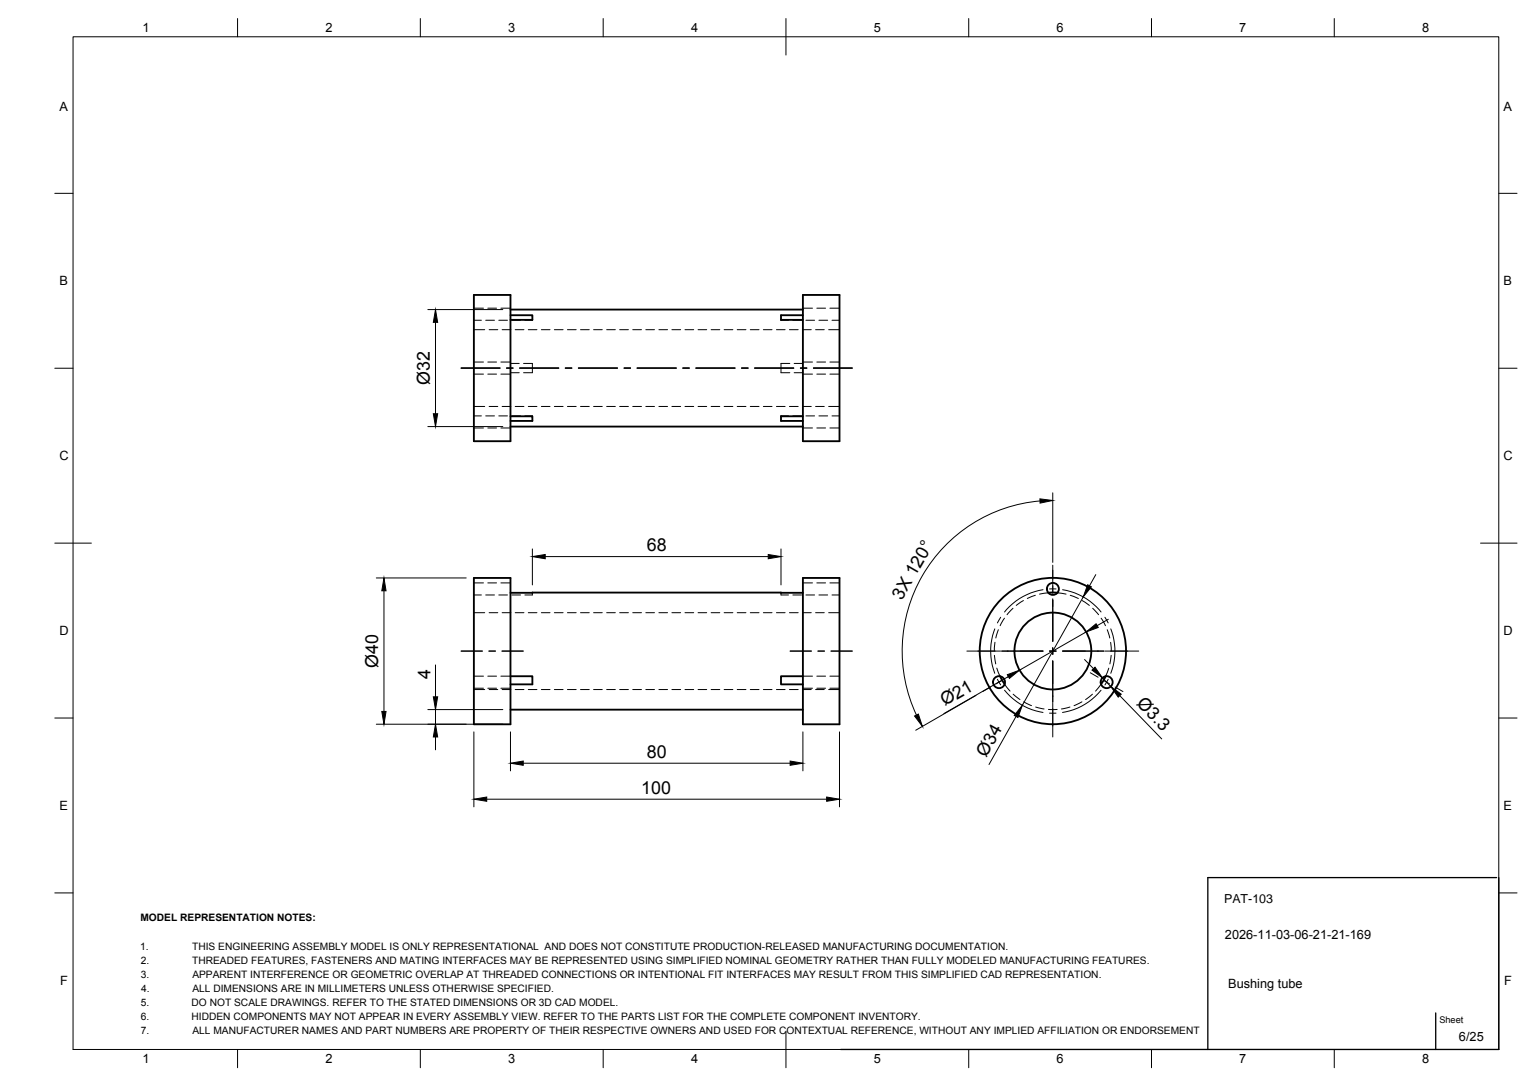
ISO-10303-21;
HEADER;
/* Generated by software containing ST-Developer
 * from STEP Tools, Inc. (www.steptools.com) 
 */

FILE_DESCRIPTION(
/* description */ ('Telescoping shaft support with lock collar'),
/* implementation_level */ '2;1');

FILE_NAME(
/* name */ 'Bushing tube.step',
/* time_stamp */ '2026-10-27T10:48:51-07:00',
/* author */ (''),
/* organization */ (''),
/* preprocessor_version */ 'ST-DEVELOPER v20.2',
/* originating_system */ 'Autodesk Translation Framework v15.17.0.0',
/* authorisation */ '');

FILE_SCHEMA (('AUTOMOTIVE_DESIGN { 1 0 10303 214 3 1 1 }'));
ENDSEC;

DATA;
#10=MECHANICAL_DESIGN_GEOMETRIC_PRESENTATION_REPRESENTATION('',(#242),#7349);
#202=SHAPE_REPRESENTATION_RELATIONSHIP('SRR','None',#7444,#222);
#222=ADVANCED_BREP_SHAPE_REPRESENTATION('',(#262),#7328);
#242=STYLED_ITEM('',(#7641),#262);
#262=MANIFOLD_SOLID_BREP('Body1',#3965);
#287=FACE_BOUND('',#746,.T.);
#288=FACE_BOUND('',#756,.T.);
#289=FACE_BOUND('',#760,.T.);
#290=FACE_BOUND('',#761,.T.);
#291=FACE_BOUND('',#762,.T.);
#292=FACE_BOUND('',#763,.T.);
#293=FACE_BOUND('',#765,.T.);
#294=FACE_BOUND('',#766,.T.);
#295=FACE_BOUND('',#767,.T.);
#296=FACE_BOUND('',#768,.T.);
#365=PLANE('',#4234);
#366=PLANE('',#4242);
#367=PLANE('',#4249);
#368=PLANE('',#4251);
#369=PLANE('',#4256);
#370=PLANE('',#4264);
#371=PLANE('',#4271);
#372=PLANE('',#4284);
#373=PLANE('',#4291);
#374=PLANE('',#4292);
#505=FACE_OUTER_BOUND('',#739,.T.);
#506=FACE_OUTER_BOUND('',#740,.T.);
#507=FACE_OUTER_BOUND('',#741,.T.);
#508=FACE_OUTER_BOUND('',#742,.T.);
#509=FACE_OUTER_BOUND('',#743,.T.);
#510=FACE_OUTER_BOUND('',#744,.T.);
#511=FACE_OUTER_BOUND('',#745,.T.);
#512=FACE_OUTER_BOUND('',#747,.T.);
#513=FACE_OUTER_BOUND('',#748,.T.);
#514=FACE_OUTER_BOUND('',#749,.T.);
#515=FACE_OUTER_BOUND('',#750,.T.);
#516=FACE_OUTER_BOUND('',#751,.T.);
#517=FACE_OUTER_BOUND('',#752,.T.);
#518=FACE_OUTER_BOUND('',#753,.T.);
#519=FACE_OUTER_BOUND('',#754,.T.);
#520=FACE_OUTER_BOUND('',#755,.T.);
#521=FACE_OUTER_BOUND('',#757,.T.);
#522=FACE_OUTER_BOUND('',#758,.T.);
#523=FACE_OUTER_BOUND('',#759,.T.);
#524=FACE_OUTER_BOUND('',#764,.T.);
#739=EDGE_LOOP('',(#2690,#2691,#2692,#2693,#2694,#2695,#2696,#2697));
#740=EDGE_LOOP('',(#2698,#2699,#2700));
#741=EDGE_LOOP('',(#2701,#2702,#2703,#2704,#2705,#2706,#2707,#2708));
#742=EDGE_LOOP('',(#2709,#2710));
#743=EDGE_LOOP('',(#2711,#2712,#2713,#2714,#2715,#2716,#2717,#2718));
#744=EDGE_LOOP('',(#2719,#2720));
#745=EDGE_LOOP('',(#2721));
#746=EDGE_LOOP('',(#2722,#2723,#2724,#2725,#2726,#2727,#2728,#2729,#2730));
#747=EDGE_LOOP('',(#2731,#2732,#2733));
#748=EDGE_LOOP('',(#2734,#2735,#2736,#2737,#2738,#2739,#2740,#2741));
#749=EDGE_LOOP('',(#2742,#2743));
#750=EDGE_LOOP('',(#2744,#2745,#2746,#2747,#2748,#2749,#2750,#2751));
#751=EDGE_LOOP('',(#2752,#2753));
#752=EDGE_LOOP('',(#2754,#2755,#2756,#2757,#2758,#2759,#2760,#2761));
#753=EDGE_LOOP('',(#2762,#2763,#2764,#2765,#2766,#2767,#2768,#2769,#2770,
#2771,#2772,#2773,#2774,#2775,#2776,#2777,#2778,#2779,#2780,#2781,#2782,
#2783,#2784,#2785,#2786,#2787,#2788,#2789));
#754=EDGE_LOOP('',(#2790,#2791,#2792,#2793));
#755=EDGE_LOOP('',(#2794));
#756=EDGE_LOOP('',(#2795,#2796,#2797,#2798,#2799,#2800,#2801,#2802,#2803));
#757=EDGE_LOOP('',(#2804,#2805,#2806,#2807));
#758=EDGE_LOOP('',(#2808,#2809,#2810,#2811));
#759=EDGE_LOOP('',(#2812));
#760=EDGE_LOOP('',(#2813));
#761=EDGE_LOOP('',(#2814));
#762=EDGE_LOOP('',(#2815));
#763=EDGE_LOOP('',(#2816));
#764=EDGE_LOOP('',(#2817));
#765=EDGE_LOOP('',(#2818));
#766=EDGE_LOOP('',(#2819));
#767=EDGE_LOOP('',(#2820));
#768=EDGE_LOOP('',(#2821));
#1043=LINE('',#6044,#1323);
#1044=LINE('',#6048,#1324);
#1045=LINE('',#6052,#1325);
#1046=LINE('',#6062,#1326);
#1047=LINE('',#6066,#1327);
#1048=LINE('',#6070,#1328);
#1049=LINE('',#6078,#1329);
#1050=LINE('',#6082,#1330);
#1051=LINE('',#6086,#1331);
#1052=LINE('',#6108,#1332);
#1053=LINE('',#6111,#1333);
#1054=LINE('',#6113,#1334);
#1055=LINE('',#6124,#1335);
#1056=LINE('',#6127,#1336);
#1057=LINE('',#6129,#1337);
#1058=LINE('',#6140,#1338);
#1059=LINE('',#6143,#1339);
#1060=LINE('',#6145,#1340);
#1061=LINE('',#6148,#1341);
#1062=LINE('',#6155,#1342);
#1063=LINE('',#6161,#1343);
#1064=LINE('',#6167,#1344);
#1323=VECTOR('',#4769,1.);
#1324=VECTOR('',#4772,1.);
#1325=VECTOR('',#4775,0.165);
#1326=VECTOR('',#4788,1.);
#1327=VECTOR('',#4791,1.);
#1328=VECTOR('',#4794,0.165);
#1329=VECTOR('',#4805,1.);
#1330=VECTOR('',#4808,1.);
#1331=VECTOR('',#4811,0.165);
#1332=VECTOR('',#4842,0.165);
#1333=VECTOR('',#4845,1.);
#1334=VECTOR('',#4846,1.);
#1335=VECTOR('',#4859,0.165);
#1336=VECTOR('',#4862,1.);
#1337=VECTOR('',#4863,1.);
#1338=VECTOR('',#4876,0.165);
#1339=VECTOR('',#4879,1.);
#1340=VECTOR('',#4880,1.);
#1341=VECTOR('',#4885,1.6);
#1342=VECTOR('',#4896,2.);
#1343=VECTOR('',#4903,2.);
#1344=VECTOR('',#4910,1.05);
#1595=CIRCLE('',#4230,0.165);
#1596=CIRCLE('',#4231,0.165);
#1597=CIRCLE('',#4232,0.165);
#1598=CIRCLE('',#4233,0.165);
#1599=CIRCLE('',#4235,1.6);
#1600=CIRCLE('',#4236,1.6);
#1601=CIRCLE('',#4238,0.165);
#1602=CIRCLE('',#4239,0.165);
#1603=CIRCLE('',#4240,0.165);
#1604=CIRCLE('',#4241,0.165);
#1605=CIRCLE('',#4243,1.6);
#1606=CIRCLE('',#4245,0.165);
#1607=CIRCLE('',#4246,0.165);
#1608=CIRCLE('',#4247,0.165);
#1609=CIRCLE('',#4248,0.165);
#1610=CIRCLE('',#4250,1.6);
#1611=CIRCLE('',#4252,2.);
#1612=CIRCLE('',#4253,1.6);
#1613=CIRCLE('',#4254,1.6);
#1614=CIRCLE('',#4255,1.6);
#1615=CIRCLE('',#4257,1.6);
#1616=CIRCLE('',#4258,0.165);
#1617=CIRCLE('',#4259,1.6);
#1618=CIRCLE('',#4261,0.165);
#1619=CIRCLE('',#4262,0.165);
#1620=CIRCLE('',#4263,0.165);
#1621=CIRCLE('',#4265,1.6);
#1622=CIRCLE('',#4266,0.165);
#1623=CIRCLE('',#4268,0.165);
#1624=CIRCLE('',#4269,0.165);
#1625=CIRCLE('',#4270,0.165);
#1626=CIRCLE('',#4272,1.6);
#1627=CIRCLE('',#4273,0.165);
#1628=CIRCLE('',#4275,0.165);
#1629=CIRCLE('',#4276,0.165);
#1630=CIRCLE('',#4277,0.165);
#1631=CIRCLE('',#4279,1.6);
#1632=CIRCLE('',#4280,1.6);
#1633=CIRCLE('',#4281,1.6);
#1634=CIRCLE('',#4283,2.);
#1635=CIRCLE('',#4285,2.);
#1636=CIRCLE('',#4287,2.);
#1637=CIRCLE('',#4289,1.05);
#1638=CIRCLE('',#4290,1.05);
#1814=VERTEX_POINT('',#6042);
#1815=VERTEX_POINT('',#6043);
#1816=VERTEX_POINT('',#6045);
#1817=VERTEX_POINT('',#6047);
#1818=VERTEX_POINT('',#6049);
#1819=VERTEX_POINT('',#6051);
#1820=VERTEX_POINT('',#6056);
#1821=VERTEX_POINT('',#6060);
#1822=VERTEX_POINT('',#6061);
#1823=VERTEX_POINT('',#6063);
#1824=VERTEX_POINT('',#6065);
#1825=VERTEX_POINT('',#6067);
#1826=VERTEX_POINT('',#6069);
#1827=VERTEX_POINT('',#6076);
#1828=VERTEX_POINT('',#6077);
#1829=VERTEX_POINT('',#6079);
#1830=VERTEX_POINT('',#6081);
#1831=VERTEX_POINT('',#6083);
#1832=VERTEX_POINT('',#6085);
#1833=VERTEX_POINT('',#6092);
#1834=VERTEX_POINT('',#6098);
#1835=VERTEX_POINT('',#6099);
#1836=VERTEX_POINT('',#6101);
#1837=VERTEX_POINT('',#6105);
#1838=VERTEX_POINT('',#6107);
#1839=VERTEX_POINT('',#6109);
#1840=VERTEX_POINT('',#6112);
#1841=VERTEX_POINT('',#6116);
#1842=VERTEX_POINT('',#6117);
#1843=VERTEX_POINT('',#6121);
#1844=VERTEX_POINT('',#6123);
#1845=VERTEX_POINT('',#6125);
#1846=VERTEX_POINT('',#6128);
#1847=VERTEX_POINT('',#6132);
#1848=VERTEX_POINT('',#6133);
#1849=VERTEX_POINT('',#6137);
#1850=VERTEX_POINT('',#6139);
#1851=VERTEX_POINT('',#6141);
#1852=VERTEX_POINT('',#6144);
#1853=VERTEX_POINT('',#6153);
#1854=VERTEX_POINT('',#6157);
#1855=VERTEX_POINT('',#6160);
#1856=VERTEX_POINT('',#6164);
#1857=VERTEX_POINT('',#6166);
#2157=EDGE_CURVE('',#1814,#1815,#1043,.T.);
#2158=EDGE_CURVE('',#1816,#1814,#1595,.T.);
#2159=EDGE_CURVE('',#1817,#1816,#1044,.T.);
#2160=EDGE_CURVE('',#1818,#1817,#1596,.T.);
#2161=EDGE_CURVE('',#1818,#1819,#1045,.T.);
#2162=EDGE_CURVE('',#1819,#1819,#1597,.T.);
#2163=EDGE_CURVE('',#1815,#1818,#1598,.T.);
#2164=EDGE_CURVE('',#1816,#1820,#1599,.T.);
#2165=EDGE_CURVE('',#1820,#1814,#1600,.T.);
#2166=EDGE_CURVE('',#1821,#1822,#1046,.T.);
#2167=EDGE_CURVE('',#1823,#1821,#1601,.T.);
#2168=EDGE_CURVE('',#1824,#1823,#1047,.T.);
#2169=EDGE_CURVE('',#1825,#1824,#1602,.T.);
#2170=EDGE_CURVE('',#1825,#1826,#1048,.T.);
#2171=EDGE_CURVE('',#1826,#1826,#1603,.T.);
#2172=EDGE_CURVE('',#1822,#1825,#1604,.T.);
#2173=EDGE_CURVE('',#1823,#1821,#1605,.T.);
#2174=EDGE_CURVE('',#1827,#1828,#1049,.T.);
#2175=EDGE_CURVE('',#1829,#1827,#1606,.T.);
#2176=EDGE_CURVE('',#1830,#1829,#1050,.T.);
#2177=EDGE_CURVE('',#1831,#1830,#1607,.T.);
#2178=EDGE_CURVE('',#1831,#1832,#1051,.T.);
#2179=EDGE_CURVE('',#1832,#1832,#1608,.T.);
#2180=EDGE_CURVE('',#1828,#1831,#1609,.T.);
#2181=EDGE_CURVE('',#1829,#1827,#1610,.T.);
#2182=EDGE_CURVE('',#1833,#1833,#1611,.T.);
#2183=EDGE_CURVE('',#1822,#1817,#1612,.T.);
#2184=EDGE_CURVE('',#1828,#1824,#1613,.T.);
#2185=EDGE_CURVE('',#1815,#1830,#1614,.T.);
#2186=EDGE_CURVE('',#1834,#1835,#1615,.T.);
#2187=EDGE_CURVE('',#1836,#1834,#1616,.T.);
#2188=EDGE_CURVE('',#1835,#1836,#1617,.T.);
#2189=EDGE_CURVE('',#1837,#1837,#1618,.T.);
#2190=EDGE_CURVE('',#1837,#1838,#1052,.T.);
#2191=EDGE_CURVE('',#1839,#1838,#1619,.T.);
#2192=EDGE_CURVE('',#1836,#1839,#1053,.T.);
#2193=EDGE_CURVE('',#1840,#1834,#1054,.T.);
#2194=EDGE_CURVE('',#1838,#1840,#1620,.T.);
#2195=EDGE_CURVE('',#1841,#1842,#1621,.T.);
#2196=EDGE_CURVE('',#1842,#1841,#1622,.T.);
#2197=EDGE_CURVE('',#1843,#1843,#1623,.T.);
#2198=EDGE_CURVE('',#1843,#1844,#1055,.T.);
#2199=EDGE_CURVE('',#1845,#1844,#1624,.T.);
#2200=EDGE_CURVE('',#1842,#1845,#1056,.T.);
#2201=EDGE_CURVE('',#1846,#1841,#1057,.T.);
#2202=EDGE_CURVE('',#1844,#1846,#1625,.T.);
#2203=EDGE_CURVE('',#1847,#1848,#1626,.T.);
#2204=EDGE_CURVE('',#1848,#1847,#1627,.T.);
#2205=EDGE_CURVE('',#1849,#1849,#1628,.T.);
#2206=EDGE_CURVE('',#1849,#1850,#1058,.T.);
#2207=EDGE_CURVE('',#1851,#1850,#1629,.T.);
#2208=EDGE_CURVE('',#1848,#1851,#1059,.T.);
#2209=EDGE_CURVE('',#1852,#1847,#1060,.T.);
#2210=EDGE_CURVE('',#1850,#1852,#1630,.T.);
#2211=EDGE_CURVE('',#1820,#1835,#1061,.T.);
#2212=EDGE_CURVE('',#1839,#1846,#1631,.T.);
#2213=EDGE_CURVE('',#1845,#1852,#1632,.T.);
#2214=EDGE_CURVE('',#1851,#1840,#1633,.T.);
#2215=EDGE_CURVE('',#1853,#1853,#1634,.T.);
#2216=EDGE_CURVE('',#1853,#1833,#1062,.T.);
#2217=EDGE_CURVE('',#1854,#1854,#1635,.T.);
#2218=EDGE_CURVE('',#1854,#1855,#1063,.T.);
#2219=EDGE_CURVE('',#1855,#1855,#1636,.T.);
#2220=EDGE_CURVE('',#1856,#1856,#1637,.T.);
#2221=EDGE_CURVE('',#1856,#1857,#1064,.T.);
#2222=EDGE_CURVE('',#1857,#1857,#1638,.T.);
#2690=ORIENTED_EDGE('',*,*,#2157,.F.);
#2691=ORIENTED_EDGE('',*,*,#2158,.F.);
#2692=ORIENTED_EDGE('',*,*,#2159,.F.);
#2693=ORIENTED_EDGE('',*,*,#2160,.F.);
#2694=ORIENTED_EDGE('',*,*,#2161,.T.);
#2695=ORIENTED_EDGE('',*,*,#2162,.F.);
#2696=ORIENTED_EDGE('',*,*,#2161,.F.);
#2697=ORIENTED_EDGE('',*,*,#2163,.F.);
#2698=ORIENTED_EDGE('',*,*,#2164,.F.);
#2699=ORIENTED_EDGE('',*,*,#2158,.T.);
#2700=ORIENTED_EDGE('',*,*,#2165,.F.);
#2701=ORIENTED_EDGE('',*,*,#2166,.F.);
#2702=ORIENTED_EDGE('',*,*,#2167,.F.);
#2703=ORIENTED_EDGE('',*,*,#2168,.F.);
#2704=ORIENTED_EDGE('',*,*,#2169,.F.);
#2705=ORIENTED_EDGE('',*,*,#2170,.T.);
#2706=ORIENTED_EDGE('',*,*,#2171,.F.);
#2707=ORIENTED_EDGE('',*,*,#2170,.F.);
#2708=ORIENTED_EDGE('',*,*,#2172,.F.);
#2709=ORIENTED_EDGE('',*,*,#2173,.F.);
#2710=ORIENTED_EDGE('',*,*,#2167,.T.);
#2711=ORIENTED_EDGE('',*,*,#2174,.F.);
#2712=ORIENTED_EDGE('',*,*,#2175,.F.);
#2713=ORIENTED_EDGE('',*,*,#2176,.F.);
#2714=ORIENTED_EDGE('',*,*,#2177,.F.);
#2715=ORIENTED_EDGE('',*,*,#2178,.T.);
#2716=ORIENTED_EDGE('',*,*,#2179,.F.);
#2717=ORIENTED_EDGE('',*,*,#2178,.F.);
#2718=ORIENTED_EDGE('',*,*,#2180,.F.);
#2719=ORIENTED_EDGE('',*,*,#2181,.F.);
#2720=ORIENTED_EDGE('',*,*,#2175,.T.);
#2721=ORIENTED_EDGE('',*,*,#2182,.F.);
#2722=ORIENTED_EDGE('',*,*,#2163,.T.);
#2723=ORIENTED_EDGE('',*,*,#2160,.T.);
#2724=ORIENTED_EDGE('',*,*,#2183,.F.);
#2725=ORIENTED_EDGE('',*,*,#2172,.T.);
#2726=ORIENTED_EDGE('',*,*,#2169,.T.);
#2727=ORIENTED_EDGE('',*,*,#2184,.F.);
#2728=ORIENTED_EDGE('',*,*,#2180,.T.);
#2729=ORIENTED_EDGE('',*,*,#2177,.T.);
#2730=ORIENTED_EDGE('',*,*,#2185,.F.);
#2731=ORIENTED_EDGE('',*,*,#2186,.F.);
#2732=ORIENTED_EDGE('',*,*,#2187,.F.);
#2733=ORIENTED_EDGE('',*,*,#2188,.F.);
#2734=ORIENTED_EDGE('',*,*,#2189,.F.);
#2735=ORIENTED_EDGE('',*,*,#2190,.T.);
#2736=ORIENTED_EDGE('',*,*,#2191,.F.);
#2737=ORIENTED_EDGE('',*,*,#2192,.F.);
#2738=ORIENTED_EDGE('',*,*,#2187,.T.);
#2739=ORIENTED_EDGE('',*,*,#2193,.F.);
#2740=ORIENTED_EDGE('',*,*,#2194,.F.);
#2741=ORIENTED_EDGE('',*,*,#2190,.F.);
#2742=ORIENTED_EDGE('',*,*,#2195,.F.);
#2743=ORIENTED_EDGE('',*,*,#2196,.F.);
#2744=ORIENTED_EDGE('',*,*,#2197,.F.);
#2745=ORIENTED_EDGE('',*,*,#2198,.T.);
#2746=ORIENTED_EDGE('',*,*,#2199,.F.);
#2747=ORIENTED_EDGE('',*,*,#2200,.F.);
#2748=ORIENTED_EDGE('',*,*,#2196,.T.);
#2749=ORIENTED_EDGE('',*,*,#2201,.F.);
#2750=ORIENTED_EDGE('',*,*,#2202,.F.);
#2751=ORIENTED_EDGE('',*,*,#2198,.F.);
#2752=ORIENTED_EDGE('',*,*,#2203,.F.);
#2753=ORIENTED_EDGE('',*,*,#2204,.F.);
#2754=ORIENTED_EDGE('',*,*,#2205,.F.);
#2755=ORIENTED_EDGE('',*,*,#2206,.T.);
#2756=ORIENTED_EDGE('',*,*,#2207,.F.);
#2757=ORIENTED_EDGE('',*,*,#2208,.F.);
#2758=ORIENTED_EDGE('',*,*,#2204,.T.);
#2759=ORIENTED_EDGE('',*,*,#2209,.F.);
#2760=ORIENTED_EDGE('',*,*,#2210,.F.);
#2761=ORIENTED_EDGE('',*,*,#2206,.F.);
#2762=ORIENTED_EDGE('',*,*,#2157,.T.);
#2763=ORIENTED_EDGE('',*,*,#2185,.T.);
#2764=ORIENTED_EDGE('',*,*,#2176,.T.);
#2765=ORIENTED_EDGE('',*,*,#2181,.T.);
#2766=ORIENTED_EDGE('',*,*,#2174,.T.);
#2767=ORIENTED_EDGE('',*,*,#2184,.T.);
#2768=ORIENTED_EDGE('',*,*,#2168,.T.);
#2769=ORIENTED_EDGE('',*,*,#2173,.T.);
#2770=ORIENTED_EDGE('',*,*,#2166,.T.);
#2771=ORIENTED_EDGE('',*,*,#2183,.T.);
#2772=ORIENTED_EDGE('',*,*,#2159,.T.);
#2773=ORIENTED_EDGE('',*,*,#2164,.T.);
#2774=ORIENTED_EDGE('',*,*,#2211,.T.);
#2775=ORIENTED_EDGE('',*,*,#2188,.T.);
#2776=ORIENTED_EDGE('',*,*,#2192,.T.);
#2777=ORIENTED_EDGE('',*,*,#2212,.T.);
#2778=ORIENTED_EDGE('',*,*,#2201,.T.);
#2779=ORIENTED_EDGE('',*,*,#2195,.T.);
#2780=ORIENTED_EDGE('',*,*,#2200,.T.);
#2781=ORIENTED_EDGE('',*,*,#2213,.T.);
#2782=ORIENTED_EDGE('',*,*,#2209,.T.);
#2783=ORIENTED_EDGE('',*,*,#2203,.T.);
#2784=ORIENTED_EDGE('',*,*,#2208,.T.);
#2785=ORIENTED_EDGE('',*,*,#2214,.T.);
#2786=ORIENTED_EDGE('',*,*,#2193,.T.);
#2787=ORIENTED_EDGE('',*,*,#2186,.T.);
#2788=ORIENTED_EDGE('',*,*,#2211,.F.);
#2789=ORIENTED_EDGE('',*,*,#2165,.T.);
#2790=ORIENTED_EDGE('',*,*,#2215,.F.);
#2791=ORIENTED_EDGE('',*,*,#2216,.T.);
#2792=ORIENTED_EDGE('',*,*,#2182,.T.);
#2793=ORIENTED_EDGE('',*,*,#2216,.F.);
#2794=ORIENTED_EDGE('',*,*,#2217,.T.);
#2795=ORIENTED_EDGE('',*,*,#2191,.T.);
#2796=ORIENTED_EDGE('',*,*,#2194,.T.);
#2797=ORIENTED_EDGE('',*,*,#2214,.F.);
#2798=ORIENTED_EDGE('',*,*,#2207,.T.);
#2799=ORIENTED_EDGE('',*,*,#2210,.T.);
#2800=ORIENTED_EDGE('',*,*,#2213,.F.);
#2801=ORIENTED_EDGE('',*,*,#2199,.T.);
#2802=ORIENTED_EDGE('',*,*,#2202,.T.);
#2803=ORIENTED_EDGE('',*,*,#2212,.F.);
#2804=ORIENTED_EDGE('',*,*,#2217,.F.);
#2805=ORIENTED_EDGE('',*,*,#2218,.T.);
#2806=ORIENTED_EDGE('',*,*,#2219,.T.);
#2807=ORIENTED_EDGE('',*,*,#2218,.F.);
#2808=ORIENTED_EDGE('',*,*,#2220,.F.);
#2809=ORIENTED_EDGE('',*,*,#2221,.T.);
#2810=ORIENTED_EDGE('',*,*,#2222,.T.);
#2811=ORIENTED_EDGE('',*,*,#2221,.F.);
#2812=ORIENTED_EDGE('',*,*,#2215,.T.);
#2813=ORIENTED_EDGE('',*,*,#2162,.T.);
#2814=ORIENTED_EDGE('',*,*,#2171,.T.);
#2815=ORIENTED_EDGE('',*,*,#2179,.T.);
#2816=ORIENTED_EDGE('',*,*,#2220,.T.);
#2817=ORIENTED_EDGE('',*,*,#2219,.F.);
#2818=ORIENTED_EDGE('',*,*,#2189,.T.);
#2819=ORIENTED_EDGE('',*,*,#2197,.T.);
#2820=ORIENTED_EDGE('',*,*,#2205,.T.);
#2821=ORIENTED_EDGE('',*,*,#2222,.F.);
#3664=CYLINDRICAL_SURFACE('',#4229,0.165);
#3665=CYLINDRICAL_SURFACE('',#4237,0.165);
#3666=CYLINDRICAL_SURFACE('',#4244,0.165);
#3667=CYLINDRICAL_SURFACE('',#4260,0.165);
#3668=CYLINDRICAL_SURFACE('',#4267,0.165);
#3669=CYLINDRICAL_SURFACE('',#4274,0.165);
#3670=CYLINDRICAL_SURFACE('',#4278,1.6);
#3671=CYLINDRICAL_SURFACE('',#4282,2.);
#3672=CYLINDRICAL_SURFACE('',#4286,2.);
#3673=CYLINDRICAL_SURFACE('',#4288,1.05);
#3748=ADVANCED_FACE('',(#505),#3664,.F.);
#3749=ADVANCED_FACE('',(#506),#365,.T.);
#3750=ADVANCED_FACE('',(#507),#3665,.F.);
#3751=ADVANCED_FACE('',(#508),#366,.T.);
#3752=ADVANCED_FACE('',(#509),#3666,.F.);
#3753=ADVANCED_FACE('',(#510),#367,.T.);
#3754=ADVANCED_FACE('',(#511,#287),#368,.F.);
#3755=ADVANCED_FACE('',(#512),#369,.F.);
#3756=ADVANCED_FACE('',(#513),#3667,.F.);
#3757=ADVANCED_FACE('',(#514),#370,.F.);
#3758=ADVANCED_FACE('',(#515),#3668,.F.);
#3759=ADVANCED_FACE('',(#516),#371,.F.);
#3760=ADVANCED_FACE('',(#517),#3669,.F.);
#3761=ADVANCED_FACE('',(#518),#3670,.T.);
#3762=ADVANCED_FACE('',(#519),#3671,.T.);
#3763=ADVANCED_FACE('',(#520,#288),#372,.T.);
#3764=ADVANCED_FACE('',(#521),#3672,.T.);
#3765=ADVANCED_FACE('',(#522),#3673,.F.);
#3766=ADVANCED_FACE('',(#523,#289,#290,#291,#292),#373,.T.);
#3767=ADVANCED_FACE('',(#524,#293,#294,#295,#296),#374,.F.);
#3965=CLOSED_SHELL('',(#3748,#3749,#3750,#3751,#3752,#3753,#3754,#3755,
#3756,#3757,#3758,#3759,#3760,#3761,#3762,#3763,#3764,#3765,#3766,#3767));
#4228=AXIS2_PLACEMENT_3D('',#6040,#4765,#4766);
#4229=AXIS2_PLACEMENT_3D('',#6041,#4767,#4768);
#4230=AXIS2_PLACEMENT_3D('',#6046,#4770,#4771);
#4231=AXIS2_PLACEMENT_3D('',#6050,#4773,#4774);
#4232=AXIS2_PLACEMENT_3D('',#6053,#4776,#4777);
#4233=AXIS2_PLACEMENT_3D('',#6054,#4778,#4779);
#4234=AXIS2_PLACEMENT_3D('',#6055,#4780,#4781);
#4235=AXIS2_PLACEMENT_3D('',#6057,#4782,#4783);
#4236=AXIS2_PLACEMENT_3D('',#6058,#4784,#4785);
#4237=AXIS2_PLACEMENT_3D('',#6059,#4786,#4787);
#4238=AXIS2_PLACEMENT_3D('',#6064,#4789,#4790);
#4239=AXIS2_PLACEMENT_3D('',#6068,#4792,#4793);
#4240=AXIS2_PLACEMENT_3D('',#6071,#4795,#4796);
#4241=AXIS2_PLACEMENT_3D('',#6072,#4797,#4798);
#4242=AXIS2_PLACEMENT_3D('',#6073,#4799,#4800);
#4243=AXIS2_PLACEMENT_3D('',#6074,#4801,#4802);
#4244=AXIS2_PLACEMENT_3D('',#6075,#4803,#4804);
#4245=AXIS2_PLACEMENT_3D('',#6080,#4806,#4807);
#4246=AXIS2_PLACEMENT_3D('',#6084,#4809,#4810);
#4247=AXIS2_PLACEMENT_3D('',#6087,#4812,#4813);
#4248=AXIS2_PLACEMENT_3D('',#6088,#4814,#4815);
#4249=AXIS2_PLACEMENT_3D('',#6089,#4816,#4817);
#4250=AXIS2_PLACEMENT_3D('',#6090,#4818,#4819);
#4251=AXIS2_PLACEMENT_3D('',#6091,#4820,#4821);
#4252=AXIS2_PLACEMENT_3D('',#6093,#4822,#4823);
#4253=AXIS2_PLACEMENT_3D('',#6094,#4824,#4825);
#4254=AXIS2_PLACEMENT_3D('',#6095,#4826,#4827);
#4255=AXIS2_PLACEMENT_3D('',#6096,#4828,#4829);
#4256=AXIS2_PLACEMENT_3D('',#6097,#4830,#4831);
#4257=AXIS2_PLACEMENT_3D('',#6100,#4832,#4833);
#4258=AXIS2_PLACEMENT_3D('',#6102,#4834,#4835);
#4259=AXIS2_PLACEMENT_3D('',#6103,#4836,#4837);
#4260=AXIS2_PLACEMENT_3D('',#6104,#4838,#4839);
#4261=AXIS2_PLACEMENT_3D('',#6106,#4840,#4841);
#4262=AXIS2_PLACEMENT_3D('',#6110,#4843,#4844);
#4263=AXIS2_PLACEMENT_3D('',#6114,#4847,#4848);
#4264=AXIS2_PLACEMENT_3D('',#6115,#4849,#4850);
#4265=AXIS2_PLACEMENT_3D('',#6118,#4851,#4852);
#4266=AXIS2_PLACEMENT_3D('',#6119,#4853,#4854);
#4267=AXIS2_PLACEMENT_3D('',#6120,#4855,#4856);
#4268=AXIS2_PLACEMENT_3D('',#6122,#4857,#4858);
#4269=AXIS2_PLACEMENT_3D('',#6126,#4860,#4861);
#4270=AXIS2_PLACEMENT_3D('',#6130,#4864,#4865);
#4271=AXIS2_PLACEMENT_3D('',#6131,#4866,#4867);
#4272=AXIS2_PLACEMENT_3D('',#6134,#4868,#4869);
#4273=AXIS2_PLACEMENT_3D('',#6135,#4870,#4871);
#4274=AXIS2_PLACEMENT_3D('',#6136,#4872,#4873);
#4275=AXIS2_PLACEMENT_3D('',#6138,#4874,#4875);
#4276=AXIS2_PLACEMENT_3D('',#6142,#4877,#4878);
#4277=AXIS2_PLACEMENT_3D('',#6146,#4881,#4882);
#4278=AXIS2_PLACEMENT_3D('',#6147,#4883,#4884);
#4279=AXIS2_PLACEMENT_3D('',#6149,#4886,#4887);
#4280=AXIS2_PLACEMENT_3D('',#6150,#4888,#4889);
#4281=AXIS2_PLACEMENT_3D('',#6151,#4890,#4891);
#4282=AXIS2_PLACEMENT_3D('',#6152,#4892,#4893);
#4283=AXIS2_PLACEMENT_3D('',#6154,#4894,#4895);
#4284=AXIS2_PLACEMENT_3D('',#6156,#4897,#4898);
#4285=AXIS2_PLACEMENT_3D('',#6158,#4899,#4900);
#4286=AXIS2_PLACEMENT_3D('',#6159,#4901,#4902);
#4287=AXIS2_PLACEMENT_3D('',#6162,#4904,#4905);
#4288=AXIS2_PLACEMENT_3D('',#6163,#4906,#4907);
#4289=AXIS2_PLACEMENT_3D('',#6165,#4908,#4909);
#4290=AXIS2_PLACEMENT_3D('',#6168,#4911,#4912);
#4291=AXIS2_PLACEMENT_3D('',#6169,#4913,#4914);
#4292=AXIS2_PLACEMENT_3D('',#6170,#4915,#4916);
#4765=DIRECTION('axis',(0.,0.,1.));
#4766=DIRECTION('refdir',(1.,0.,0.));
#4767=DIRECTION('center_axis',(1.,0.,0.));
#4768=DIRECTION('ref_axis',(0.,0.,-1.));
#4769=DIRECTION('',(1.,0.,0.));
#4770=DIRECTION('center_axis',(1.,0.,0.));
#4771=DIRECTION('ref_axis',(0.,0.,-1.));
#4772=DIRECTION('',(-1.,0.,0.));
#4773=DIRECTION('center_axis',(1.,0.,0.));
#4774=DIRECTION('ref_axis',(0.,0.,-1.));
#4775=DIRECTION('',(1.,0.,0.));
#4776=DIRECTION('center_axis',(-1.,0.,0.));
#4777=DIRECTION('ref_axis',(0.,0.,-1.));
#4778=DIRECTION('center_axis',(1.,0.,0.));
#4779=DIRECTION('ref_axis',(0.,0.,-1.));
#4780=DIRECTION('center_axis',(1.,0.,0.));
#4781=DIRECTION('ref_axis',(0.,0.,-1.));
#4782=DIRECTION('center_axis',(-1.,0.,0.));
#4783=DIRECTION('ref_axis',(0.,0.,-1.));
#4784=DIRECTION('center_axis',(-1.,0.,0.));
#4785=DIRECTION('ref_axis',(0.,0.,-1.));
#4786=DIRECTION('center_axis',(1.,0.,0.));
#4787=DIRECTION('ref_axis',(0.,0.,-1.));
#4788=DIRECTION('',(1.,0.,0.));
#4789=DIRECTION('center_axis',(1.,0.,0.));
#4790=DIRECTION('ref_axis',(0.,0.,-1.));
#4791=DIRECTION('',(-1.,0.,0.));
#4792=DIRECTION('center_axis',(1.,0.,0.));
#4793=DIRECTION('ref_axis',(0.,0.,-1.));
#4794=DIRECTION('',(1.,0.,0.));
#4795=DIRECTION('center_axis',(-1.,0.,0.));
#4796=DIRECTION('ref_axis',(0.,0.,-1.));
#4797=DIRECTION('center_axis',(1.,0.,0.));
#4798=DIRECTION('ref_axis',(0.,0.,-1.));
#4799=DIRECTION('center_axis',(1.,0.,0.));
#4800=DIRECTION('ref_axis',(0.,0.,-1.));
#4801=DIRECTION('center_axis',(-1.,0.,0.));
#4802=DIRECTION('ref_axis',(0.,0.,-1.));
#4803=DIRECTION('center_axis',(1.,0.,0.));
#4804=DIRECTION('ref_axis',(0.,0.,-1.));
#4805=DIRECTION('',(1.,0.,0.));
#4806=DIRECTION('center_axis',(1.,0.,0.));
#4807=DIRECTION('ref_axis',(0.,0.,-1.));
#4808=DIRECTION('',(-1.,0.,0.));
#4809=DIRECTION('center_axis',(1.,0.,0.));
#4810=DIRECTION('ref_axis',(0.,0.,-1.));
#4811=DIRECTION('',(1.,0.,0.));
#4812=DIRECTION('center_axis',(-1.,0.,0.));
#4813=DIRECTION('ref_axis',(0.,0.,-1.));
#4814=DIRECTION('center_axis',(1.,0.,0.));
#4815=DIRECTION('ref_axis',(0.,0.,-1.));
#4816=DIRECTION('center_axis',(1.,0.,0.));
#4817=DIRECTION('ref_axis',(0.,0.,-1.));
#4818=DIRECTION('center_axis',(-1.,0.,0.));
#4819=DIRECTION('ref_axis',(0.,0.,-1.));
#4820=DIRECTION('center_axis',(1.,0.,0.));
#4821=DIRECTION('ref_axis',(0.,0.,-1.));
#4822=DIRECTION('center_axis',(1.,0.,0.));
#4823=DIRECTION('ref_axis',(0.,0.,-1.));
#4824=DIRECTION('center_axis',(-1.,0.,0.));
#4825=DIRECTION('ref_axis',(0.,0.,-1.));
#4826=DIRECTION('center_axis',(-1.,0.,0.));
#4827=DIRECTION('ref_axis',(0.,0.,-1.));
#4828=DIRECTION('center_axis',(-1.,0.,0.));
#4829=DIRECTION('ref_axis',(0.,0.,-1.));
#4830=DIRECTION('center_axis',(1.,0.,0.));
#4831=DIRECTION('ref_axis',(0.,0.,-1.));
#4832=DIRECTION('center_axis',(1.,0.,0.));
#4833=DIRECTION('ref_axis',(0.,0.,-1.));
#4834=DIRECTION('center_axis',(1.,0.,0.));
#4835=DIRECTION('ref_axis',(0.,0.,-1.));
#4836=DIRECTION('center_axis',(1.,0.,0.));
#4837=DIRECTION('ref_axis',(0.,0.,-1.));
#4838=DIRECTION('center_axis',(1.,0.,0.));
#4839=DIRECTION('ref_axis',(0.,0.,-1.));
#4840=DIRECTION('center_axis',(1.,0.,0.));
#4841=DIRECTION('ref_axis',(0.,0.,-1.));
#4842=DIRECTION('',(1.,0.,0.));
#4843=DIRECTION('center_axis',(-1.,0.,0.));
#4844=DIRECTION('ref_axis',(0.,0.,-1.));
#4845=DIRECTION('',(-1.,0.,0.));
#4846=DIRECTION('',(1.,0.,0.));
#4847=DIRECTION('center_axis',(-1.,0.,0.));
#4848=DIRECTION('ref_axis',(0.,0.,-1.));
#4849=DIRECTION('center_axis',(1.,0.,0.));
#4850=DIRECTION('ref_axis',(0.,0.,-1.));
#4851=DIRECTION('center_axis',(1.,0.,0.));
#4852=DIRECTION('ref_axis',(0.,0.,-1.));
#4853=DIRECTION('center_axis',(1.,0.,0.));
#4854=DIRECTION('ref_axis',(0.,0.,-1.));
#4855=DIRECTION('center_axis',(1.,0.,0.));
#4856=DIRECTION('ref_axis',(0.,0.,-1.));
#4857=DIRECTION('center_axis',(1.,0.,0.));
#4858=DIRECTION('ref_axis',(0.,0.,-1.));
#4859=DIRECTION('',(1.,0.,0.));
#4860=DIRECTION('center_axis',(-1.,0.,0.));
#4861=DIRECTION('ref_axis',(0.,0.,-1.));
#4862=DIRECTION('',(-1.,0.,0.));
#4863=DIRECTION('',(1.,0.,0.));
#4864=DIRECTION('center_axis',(-1.,0.,0.));
#4865=DIRECTION('ref_axis',(0.,0.,-1.));
#4866=DIRECTION('center_axis',(1.,0.,0.));
#4867=DIRECTION('ref_axis',(0.,0.,-1.));
#4868=DIRECTION('center_axis',(1.,0.,0.));
#4869=DIRECTION('ref_axis',(0.,0.,-1.));
#4870=DIRECTION('center_axis',(1.,0.,0.));
#4871=DIRECTION('ref_axis',(0.,0.,-1.));
#4872=DIRECTION('center_axis',(1.,0.,0.));
#4873=DIRECTION('ref_axis',(0.,0.,-1.));
#4874=DIRECTION('center_axis',(1.,0.,0.));
#4875=DIRECTION('ref_axis',(0.,0.,-1.));
#4876=DIRECTION('',(1.,0.,0.));
#4877=DIRECTION('center_axis',(-1.,0.,0.));
#4878=DIRECTION('ref_axis',(0.,0.,-1.));
#4879=DIRECTION('',(-1.,0.,0.));
#4880=DIRECTION('',(1.,0.,0.));
#4881=DIRECTION('center_axis',(-1.,0.,0.));
#4882=DIRECTION('ref_axis',(0.,0.,-1.));
#4883=DIRECTION('center_axis',(1.,0.,0.));
#4884=DIRECTION('ref_axis',(0.,0.,-1.));
#4885=DIRECTION('',(-1.,0.,0.));
#4886=DIRECTION('center_axis',(1.,0.,0.));
#4887=DIRECTION('ref_axis',(0.,0.,-1.));
#4888=DIRECTION('center_axis',(1.,0.,0.));
#4889=DIRECTION('ref_axis',(0.,0.,-1.));
#4890=DIRECTION('center_axis',(1.,0.,0.));
#4891=DIRECTION('ref_axis',(0.,0.,-1.));
#4892=DIRECTION('center_axis',(1.,0.,0.));
#4893=DIRECTION('ref_axis',(0.,0.,-1.));
#4894=DIRECTION('center_axis',(1.,0.,0.));
#4895=DIRECTION('ref_axis',(0.,0.,-1.));
#4896=DIRECTION('',(-1.,0.,0.));
#4897=DIRECTION('center_axis',(1.,0.,0.));
#4898=DIRECTION('ref_axis',(0.,0.,-1.));
#4899=DIRECTION('center_axis',(1.,0.,0.));
#4900=DIRECTION('ref_axis',(0.,0.,-1.));
#4901=DIRECTION('center_axis',(1.,0.,0.));
#4902=DIRECTION('ref_axis',(0.,0.,-1.));
#4903=DIRECTION('',(-1.,0.,0.));
#4904=DIRECTION('center_axis',(1.,0.,0.));
#4905=DIRECTION('ref_axis',(0.,0.,-1.));
#4906=DIRECTION('center_axis',(1.,0.,0.));
#4907=DIRECTION('ref_axis',(0.,0.,-1.));
#4908=DIRECTION('center_axis',(-1.,0.,0.));
#4909=DIRECTION('ref_axis',(0.,0.,-1.));
#4910=DIRECTION('',(-1.,0.,0.));
#4911=DIRECTION('center_axis',(-1.,0.,0.));
#4912=DIRECTION('ref_axis',(0.,0.,-1.));
#4913=DIRECTION('center_axis',(1.,0.,0.));
#4914=DIRECTION('ref_axis',(0.,0.,-1.));
#4915=DIRECTION('center_axis',(1.,0.,0.));
#4916=DIRECTION('ref_axis',(0.,0.,-1.));
#6040=CARTESIAN_POINT('',(0.,0.,0.));
#6041=CARTESIAN_POINT('Origin',(8.4,1.04094977927525E-16,5.2));
#6042=CARTESIAN_POINT('',(8.4,0.12722459888658,5.09493382352941));
#6043=CARTESIAN_POINT('',(9.,0.127224598886581,5.09493382352941));
#6044=CARTESIAN_POINT('',(8.4,0.12722459888658,5.09493382352941));
#6045=CARTESIAN_POINT('',(8.4,-0.12722459888658,5.09493382352941));
#6046=CARTESIAN_POINT('Origin',(8.4,1.04094977927525E-16,5.2));
#6047=CARTESIAN_POINT('',(9.,-0.127224598886581,5.09493382352941));
#6048=CARTESIAN_POINT('',(8.4,-0.12722459888658,5.09493382352941));
#6049=CARTESIAN_POINT('',(9.,8.38883057415937E-17,5.365));
#6050=CARTESIAN_POINT('Origin',(9.,1.04094977927525E-16,5.2));
#6051=CARTESIAN_POINT('',(10.,1.24301650113456E-16,5.365));
#6052=CARTESIAN_POINT('',(8.4,8.38883057415937E-17,5.365));
#6053=CARTESIAN_POINT('Origin',(10.,1.04094977927525E-16,5.2));
#6054=CARTESIAN_POINT('Origin',(9.,1.04094977927525E-16,5.2));
#6055=CARTESIAN_POINT('Origin',(8.4,1.11022302462516E-16,5.2));
#6056=CARTESIAN_POINT('',(8.4,-1.95943487863577E-16,5.1));
#6057=CARTESIAN_POINT('Origin',(8.4,0.,3.5));
#6058=CARTESIAN_POINT('Origin',(8.4,0.,3.5));
#6059=CARTESIAN_POINT('Origin',(8.4,-1.47224318643355,2.65));
#6060=CARTESIAN_POINT('',(8.4,-1.44486550797481,2.81271282285736));
#6061=CARTESIAN_POINT('',(9.,-1.44486550797481,2.81271282285736));
#6062=CARTESIAN_POINT('',(8.4,-1.44486550797481,2.81271282285736));
#6063=CARTESIAN_POINT('',(8.4,-1.31764090908823,2.59235335361323));
#6064=CARTESIAN_POINT('Origin',(8.4,-1.47224318643355,2.65));
#6065=CARTESIAN_POINT('',(9.,-1.31764090908823,2.59235335361323));
#6066=CARTESIAN_POINT('',(8.4,-1.31764090908823,2.59235335361323));
#6067=CARTESIAN_POINT('',(9.,-1.47224318643355,2.815));
#6068=CARTESIAN_POINT('Origin',(9.,-1.47224318643355,2.65));
#6069=CARTESIAN_POINT('',(10.,-1.47224318643355,2.815));
#6070=CARTESIAN_POINT('',(8.4,-1.47224318643355,2.815));
#6071=CARTESIAN_POINT('Origin',(10.,-1.47224318643355,2.65));
#6072=CARTESIAN_POINT('Origin',(9.,-1.47224318643355,2.65));
#6073=CARTESIAN_POINT('Origin',(8.4,-1.47224318643355,2.65));
#6074=CARTESIAN_POINT('Origin',(8.4,0.,3.5));
#6075=CARTESIAN_POINT('Origin',(8.4,1.47224318643355,2.65));
#6076=CARTESIAN_POINT('',(8.4,1.31764090908823,2.59235335361323));
#6077=CARTESIAN_POINT('',(9.,1.31764090908823,2.59235335361323));
#6078=CARTESIAN_POINT('',(8.4,1.31764090908823,2.59235335361323));
#6079=CARTESIAN_POINT('',(8.4,1.44486550797481,2.81271282285736));
#6080=CARTESIAN_POINT('Origin',(8.4,1.47224318643355,2.65));
#6081=CARTESIAN_POINT('',(9.,1.44486550797481,2.81271282285736));
#6082=CARTESIAN_POINT('',(8.4,1.44486550797481,2.81271282285736));
#6083=CARTESIAN_POINT('',(9.,1.47224318643355,2.815));
#6084=CARTESIAN_POINT('Origin',(9.,1.47224318643355,2.65));
#6085=CARTESIAN_POINT('',(10.,1.47224318643355,2.815));
#6086=CARTESIAN_POINT('',(8.4,1.47224318643355,2.815));
#6087=CARTESIAN_POINT('Origin',(10.,1.47224318643355,2.65));
#6088=CARTESIAN_POINT('Origin',(9.,1.47224318643355,2.65));
#6089=CARTESIAN_POINT('Origin',(8.4,1.47224318643355,2.65));
#6090=CARTESIAN_POINT('Origin',(8.4,0.,3.5));
#6091=CARTESIAN_POINT('Origin',(9.,0.,3.5));
#6092=CARTESIAN_POINT('',(9.,-2.44929359829471E-16,5.5));
#6093=CARTESIAN_POINT('Origin',(9.,0.,3.5));
#6094=CARTESIAN_POINT('Origin',(9.,0.,3.5));
#6095=CARTESIAN_POINT('Origin',(9.,0.,3.5));
#6096=CARTESIAN_POINT('Origin',(9.,0.,3.5));
#6097=CARTESIAN_POINT('Origin',(1.6,1.11022302462516E-16,5.2));
#6098=CARTESIAN_POINT('',(1.6,0.12722459888658,5.09493382352941));
#6099=CARTESIAN_POINT('',(1.6,-1.95943487863577E-16,5.1));
#6100=CARTESIAN_POINT('Origin',(1.6,0.,3.5));
#6101=CARTESIAN_POINT('',(1.6,-0.12722459888658,5.09493382352941));
#6102=CARTESIAN_POINT('Origin',(1.6,1.04094977927525E-16,5.2));
#6103=CARTESIAN_POINT('Origin',(1.6,0.,3.5));
#6104=CARTESIAN_POINT('Origin',(-0.1,1.04094977927525E-16,5.2));
#6105=CARTESIAN_POINT('',(0.,8.38883057415937E-17,5.365));
#6106=CARTESIAN_POINT('Origin',(0.,1.04094977927525E-16,5.2));
#6107=CARTESIAN_POINT('',(1.,8.38883057415937E-17,5.365));
#6108=CARTESIAN_POINT('',(-0.1,8.38883057415937E-17,5.365));
#6109=CARTESIAN_POINT('',(1.,-0.127224598886581,5.09493382352941));
#6110=CARTESIAN_POINT('Origin',(1.,1.04094977927525E-16,5.2));
#6111=CARTESIAN_POINT('',(-0.1,-0.12722459888658,5.09493382352941));
#6112=CARTESIAN_POINT('',(1.,0.127224598886581,5.09493382352941));
#6113=CARTESIAN_POINT('',(-0.1,0.12722459888658,5.09493382352941));
#6114=CARTESIAN_POINT('Origin',(1.,1.04094977927525E-16,5.2));
#6115=CARTESIAN_POINT('Origin',(1.6,-1.47224318643355,2.65));
#6116=CARTESIAN_POINT('',(1.6,-1.44486550797481,2.81271282285736));
#6117=CARTESIAN_POINT('',(1.6,-1.31764090908823,2.59235335361323));
#6118=CARTESIAN_POINT('Origin',(1.6,0.,3.5));
#6119=CARTESIAN_POINT('Origin',(1.6,-1.47224318643355,2.65));
#6120=CARTESIAN_POINT('Origin',(-0.1,-1.47224318643355,2.65));
#6121=CARTESIAN_POINT('',(0.,-1.47224318643355,2.815));
#6122=CARTESIAN_POINT('Origin',(0.,-1.47224318643355,2.65));
#6123=CARTESIAN_POINT('',(1.,-1.47224318643355,2.815));
#6124=CARTESIAN_POINT('',(-0.1,-1.47224318643355,2.815));
#6125=CARTESIAN_POINT('',(1.,-1.31764090908823,2.59235335361323));
#6126=CARTESIAN_POINT('Origin',(1.,-1.47224318643355,2.65));
#6127=CARTESIAN_POINT('',(-0.1,-1.31764090908823,2.59235335361323));
#6128=CARTESIAN_POINT('',(1.,-1.44486550797481,2.81271282285736));
#6129=CARTESIAN_POINT('',(-0.1,-1.44486550797481,2.81271282285736));
#6130=CARTESIAN_POINT('Origin',(1.,-1.47224318643355,2.65));
#6131=CARTESIAN_POINT('Origin',(1.6,1.47224318643355,2.65));
#6132=CARTESIAN_POINT('',(1.6,1.31764090908823,2.59235335361323));
#6133=CARTESIAN_POINT('',(1.6,1.44486550797481,2.81271282285736));
#6134=CARTESIAN_POINT('Origin',(1.6,0.,3.5));
#6135=CARTESIAN_POINT('Origin',(1.6,1.47224318643355,2.65));
#6136=CARTESIAN_POINT('Origin',(-0.1,1.47224318643355,2.65));
#6137=CARTESIAN_POINT('',(0.,1.47224318643355,2.815));
#6138=CARTESIAN_POINT('Origin',(0.,1.47224318643355,2.65));
#6139=CARTESIAN_POINT('',(1.,1.47224318643355,2.815));
#6140=CARTESIAN_POINT('',(-0.1,1.47224318643355,2.815));
#6141=CARTESIAN_POINT('',(1.,1.44486550797481,2.81271282285736));
#6142=CARTESIAN_POINT('Origin',(1.,1.47224318643355,2.65));
#6143=CARTESIAN_POINT('',(-0.1,1.44486550797481,2.81271282285736));
#6144=CARTESIAN_POINT('',(1.,1.31764090908823,2.59235335361323));
#6145=CARTESIAN_POINT('',(-0.1,1.31764090908823,2.59235335361323));
#6146=CARTESIAN_POINT('Origin',(1.,1.47224318643355,2.65));
#6147=CARTESIAN_POINT('Origin',(0.,0.,3.5));
#6148=CARTESIAN_POINT('',(0.,-1.95943487863577E-16,5.1));
#6149=CARTESIAN_POINT('Origin',(1.,0.,3.5));
#6150=CARTESIAN_POINT('Origin',(1.,0.,3.5));
#6151=CARTESIAN_POINT('Origin',(1.,0.,3.5));
#6152=CARTESIAN_POINT('Origin',(9.,0.,3.5));
#6153=CARTESIAN_POINT('',(10.,-2.44929359829471E-16,5.5));
#6154=CARTESIAN_POINT('Origin',(10.,0.,3.5));
#6155=CARTESIAN_POINT('',(9.,-2.44929359829471E-16,5.5));
#6156=CARTESIAN_POINT('Origin',(1.,0.,3.5));
#6157=CARTESIAN_POINT('',(1.,-2.44929359829471E-16,5.5));
#6158=CARTESIAN_POINT('Origin',(1.,0.,3.5));
#6159=CARTESIAN_POINT('Origin',(0.,0.,3.5));
#6160=CARTESIAN_POINT('',(0.,-2.44929359829471E-16,5.5));
#6161=CARTESIAN_POINT('',(0.,-2.44929359829471E-16,5.5));
#6162=CARTESIAN_POINT('Origin',(0.,0.,3.5));
#6163=CARTESIAN_POINT('Origin',(0.,0.,3.5));
#6164=CARTESIAN_POINT('',(10.,-1.28587913910472E-16,4.55));
#6165=CARTESIAN_POINT('Origin',(10.,0.,3.5));
#6166=CARTESIAN_POINT('',(0.,-1.28587913910472E-16,4.55));
#6167=CARTESIAN_POINT('',(0.,-1.28587913910472E-16,4.55));
#6168=CARTESIAN_POINT('Origin',(0.,0.,3.5));
#6169=CARTESIAN_POINT('Origin',(10.,0.,3.5));
#6170=CARTESIAN_POINT('Origin',(0.,0.,3.5));
#7303=UNCERTAINTY_MEASURE_WITH_UNIT(LENGTH_MEASURE(0.001),#7350,
'DISTANCE_ACCURACY_VALUE',
'Maximum model space distance between geometric entities at asserted c
onnectivities');
#7324=UNCERTAINTY_MEASURE_WITH_UNIT(LENGTH_MEASURE(0.001),#7350,
'DISTANCE_ACCURACY_VALUE',
'Maximum model space distance between geometric entities at asserted c
onnectivities');
#7328=(
GEOMETRIC_REPRESENTATION_CONTEXT(3)
GLOBAL_UNCERTAINTY_ASSIGNED_CONTEXT((#7303))
GLOBAL_UNIT_ASSIGNED_CONTEXT((#7350,#7352,#7353))
REPRESENTATION_CONTEXT('','3D')
);
#7349=(
GEOMETRIC_REPRESENTATION_CONTEXT(3)
GLOBAL_UNCERTAINTY_ASSIGNED_CONTEXT((#7324))
GLOBAL_UNIT_ASSIGNED_CONTEXT((#7350,#7352,#7353))
REPRESENTATION_CONTEXT('','3D')
);
#7350=(
LENGTH_UNIT()
NAMED_UNIT(*)
SI_UNIT(.CENTI.,.METRE.)
);
#7352=(
NAMED_UNIT(*)
PLANE_ANGLE_UNIT()
SI_UNIT($,.RADIAN.)
);
#7353=(
NAMED_UNIT(*)
SI_UNIT($,.STERADIAN.)
SOLID_ANGLE_UNIT()
);
#7357=SHAPE_DEFINITION_REPRESENTATION(#7381,#7444);
#7381=PRODUCT_DEFINITION_SHAPE('',$,#7469);
#7444=SHAPE_REPRESENTATION('',(#4228),#7328);
#7465=PRODUCT_DEFINITION_CONTEXT('part definition',#7539,'design');
#7469=PRODUCT_DEFINITION('Bushing tube','Bushing tube',#7493,#7465);
#7493=PRODUCT_DEFINITION_FORMATION('',$,#7544);
#7539=APPLICATION_CONTEXT(
'Core Data for Automotive Mechanical Design Process');
#7540=PRODUCT_CONTEXT('part definition',#7539,'mechanical');
#7544=PRODUCT('Bushing tube','Bushing tube','Bushing tube',(#7540));
#7635=COLOUR_RGB('Off White',0.89,0.88,0.83);
#7636=FILL_AREA_STYLE_COLOUR('',#7635);
#7637=FILL_AREA_STYLE('',(#7636));
#7638=SURFACE_STYLE_FILL_AREA(#7637);
#7639=SURFACE_SIDE_STYLE('',(#7638));
#7640=SURFACE_STYLE_USAGE(.BOTH.,#7639);
#7641=PRESENTATION_STYLE_ASSIGNMENT((#7640));
ENDSEC;
END-ISO-10303-21;
